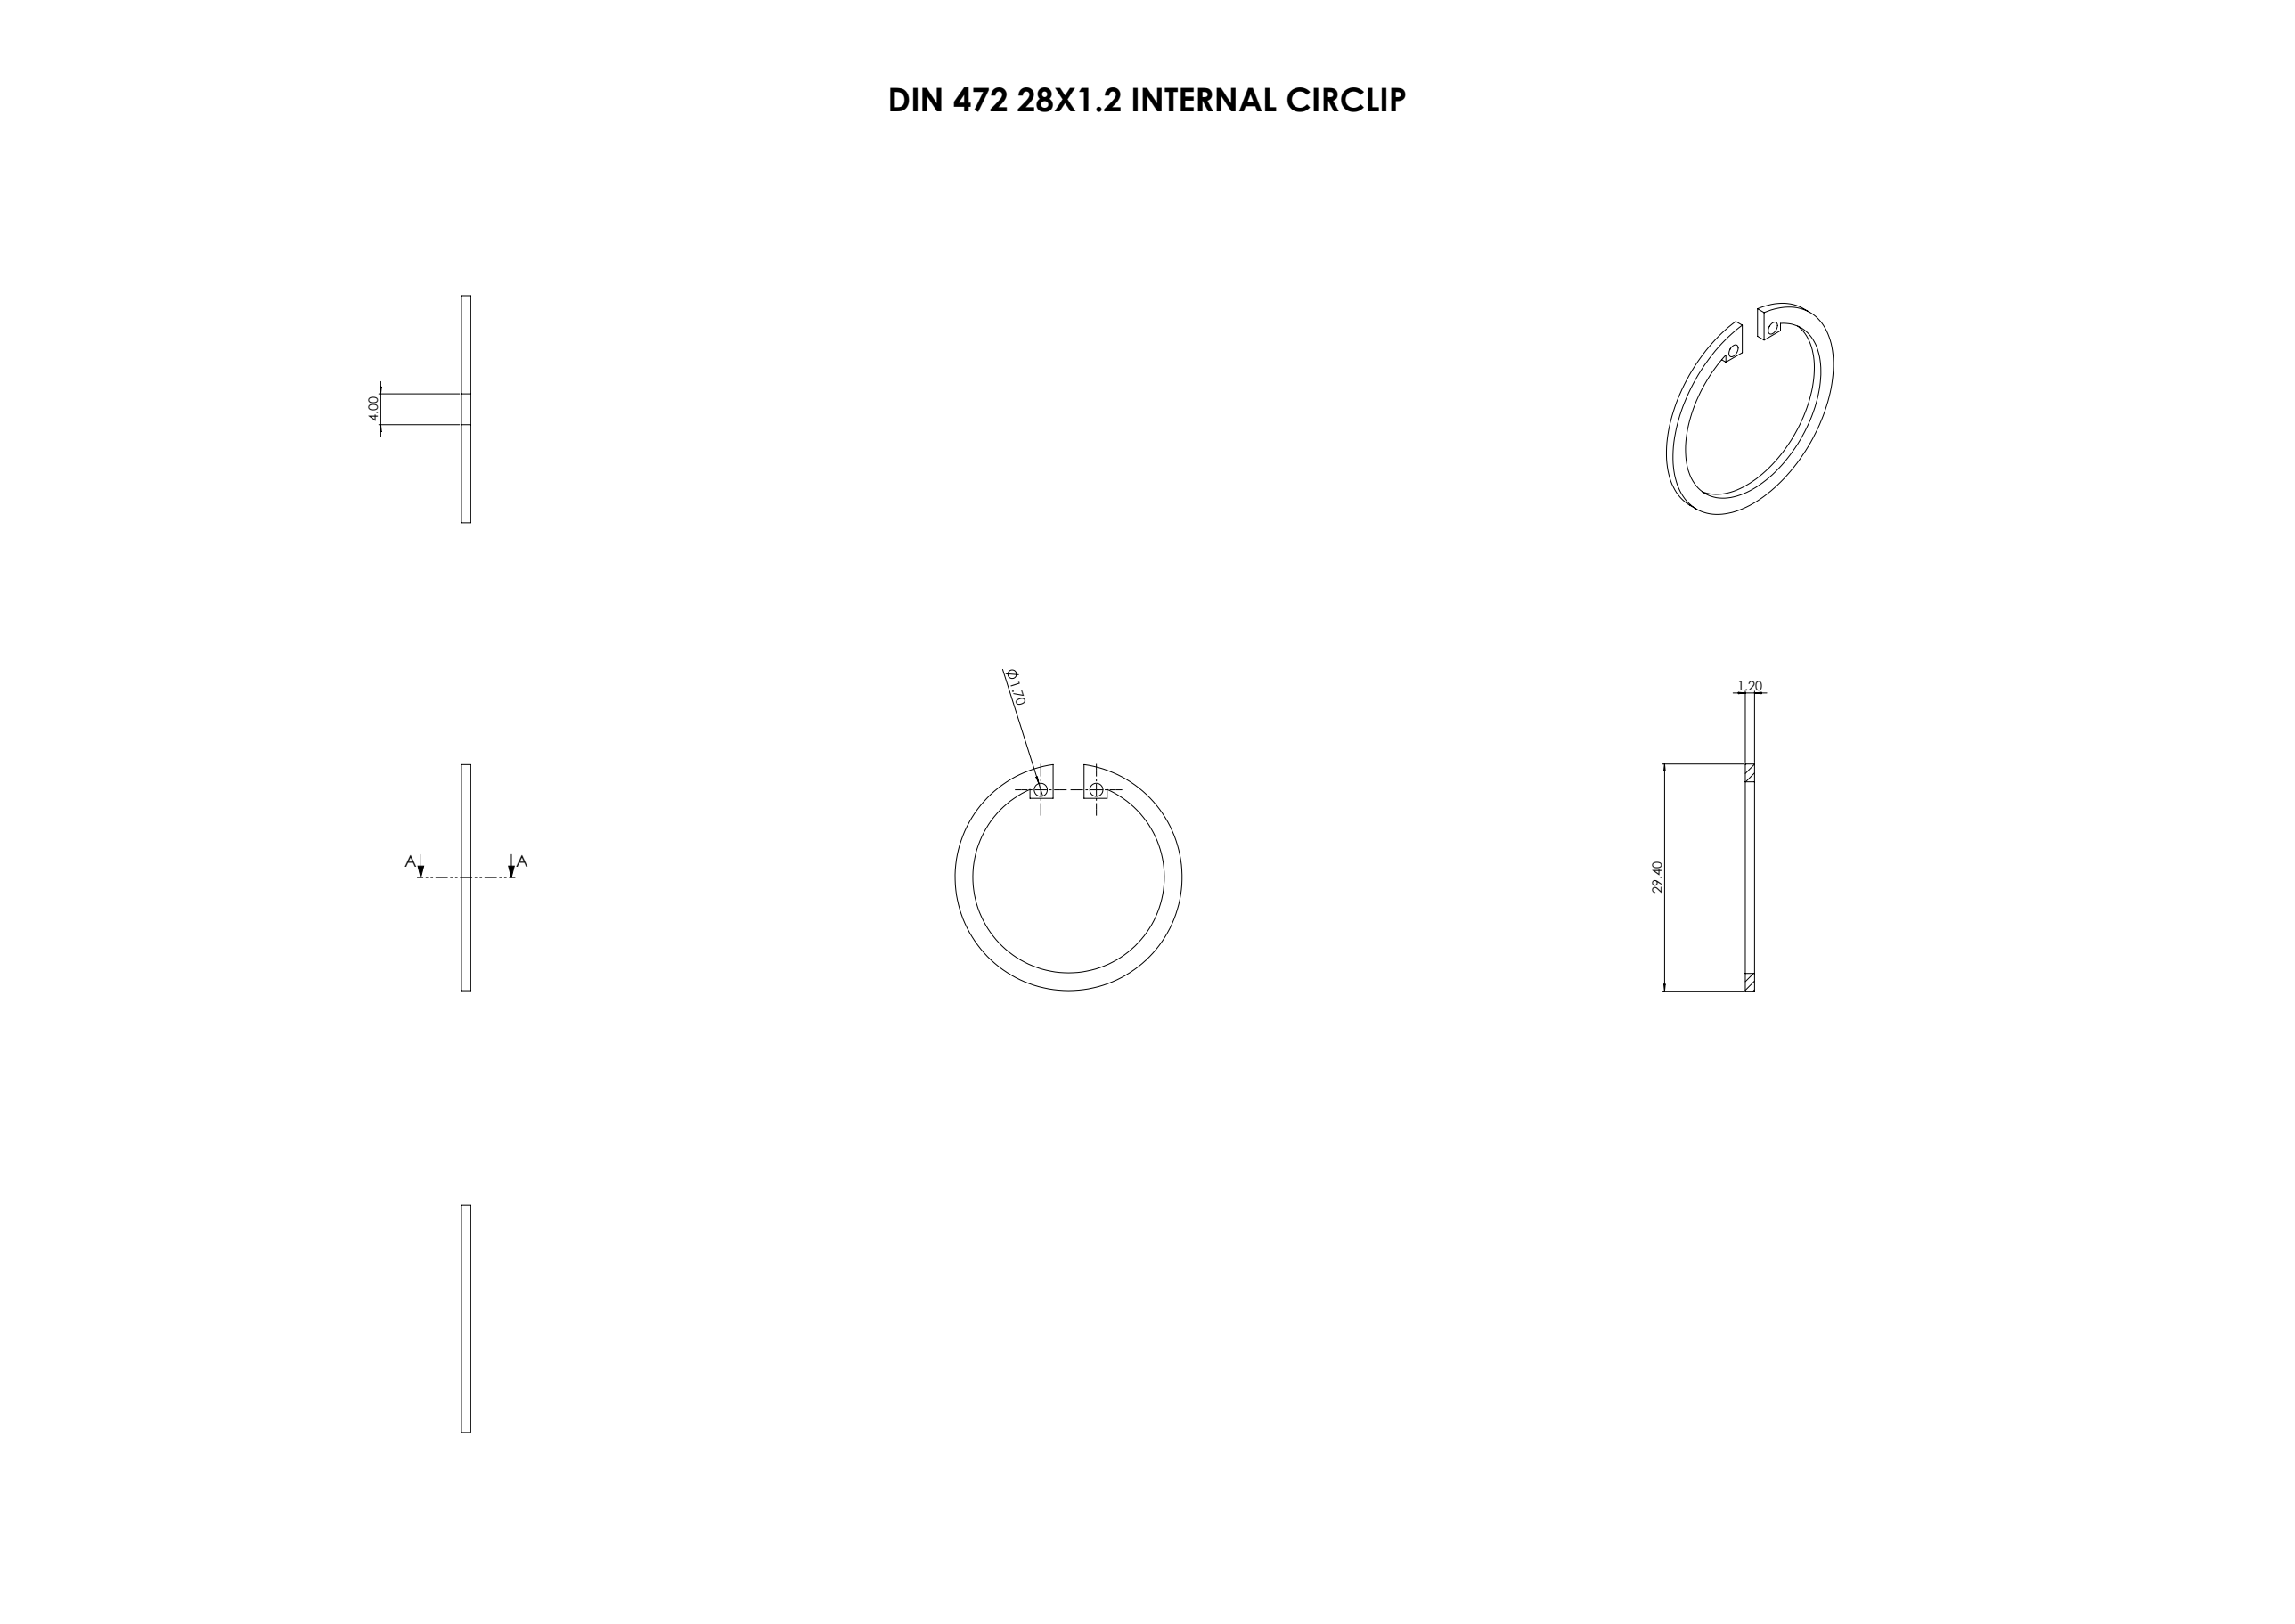
ISO-10303-21;
HEADER;
/* Generated by software containing ST-Developer
 * from STEP Tools, Inc. (www.steptools.com) 
 */

FILE_DESCRIPTION(
/* description */ (''),
/* implementation_level */ '2;1');

FILE_NAME(
/* name */ '10_DIN_472_28x1.2_Internal_Circlip.step',
/* time_stamp */ '2026-10-11T09:12:28-07:00',
/* author */ (''),
/* organization */ (''),
/* preprocessor_version */ 'ST-DEVELOPER v20.2',
/* originating_system */ 'Autodesk Translation Framework v15.15.0.0',
/* authorisation */ '');

FILE_SCHEMA (('AUTOMOTIVE_DESIGN { 1 0 10303 214 3 1 1 }'));
ENDSEC;

DATA;
#10=MECHANICAL_DESIGN_GEOMETRIC_PRESENTATION_REPRESENTATION('',(#656),#23254);
#636=SHAPE_REPRESENTATION_RELATIONSHIP('SRR','None',#23309,#646);
#646=ADVANCED_BREP_SHAPE_REPRESENTATION('',(#666),#23253);
#656=STYLED_ITEM('',(#23462),#666);
#666=MANIFOLD_SOLID_BREP('Body1',#7034);
#848=FACE_BOUND('',#1829,.T.);
#849=FACE_BOUND('',#1830,.T.);
#850=FACE_BOUND('',#1838,.T.);
#851=FACE_BOUND('',#1839,.T.);
#971=PLANE('',#7802);
#972=PLANE('',#7804);
#973=PLANE('',#7805);
#974=PLANE('',#7806);
#975=PLANE('',#7807);
#976=PLANE('',#7808);
#977=PLANE('',#7809);
#978=PLANE('',#7810);
#1362=FACE_OUTER_BOUND('',#1825,.T.);
#1363=FACE_OUTER_BOUND('',#1826,.T.);
#1364=FACE_OUTER_BOUND('',#1827,.T.);
#1365=FACE_OUTER_BOUND('',#1828,.T.);
#1366=FACE_OUTER_BOUND('',#1831,.T.);
#1367=FACE_OUTER_BOUND('',#1832,.T.);
#1368=FACE_OUTER_BOUND('',#1833,.T.);
#1369=FACE_OUTER_BOUND('',#1834,.T.);
#1370=FACE_OUTER_BOUND('',#1835,.T.);
#1371=FACE_OUTER_BOUND('',#1836,.T.);
#1372=FACE_OUTER_BOUND('',#1837,.T.);
#1373=FACE_OUTER_BOUND('',#1840,.T.);
#1825=EDGE_LOOP('',(#6507,#6508,#6509,#6510));
#1826=EDGE_LOOP('',(#6511,#6512,#6513,#6514));
#1827=EDGE_LOOP('',(#6515,#6516,#6517,#6518));
#1828=EDGE_LOOP('',(#6519,#6520,#6521,#6522,#6523,#6524,#6525,#6526));
#1829=EDGE_LOOP('',(#6527));
#1830=EDGE_LOOP('',(#6528));
#1831=EDGE_LOOP('',(#6529,#6530,#6531,#6532));
#1832=EDGE_LOOP('',(#6533,#6534,#6535,#6536));
#1833=EDGE_LOOP('',(#6537,#6538,#6539,#6540));
#1834=EDGE_LOOP('',(#6541,#6542,#6543,#6544));
#1835=EDGE_LOOP('',(#6545,#6546,#6547,#6548));
#1836=EDGE_LOOP('',(#6549,#6550,#6551,#6552));
#1837=EDGE_LOOP('',(#6553,#6554,#6555,#6556,#6557,#6558,#6559,#6560));
#1838=EDGE_LOOP('',(#6561));
#1839=EDGE_LOOP('',(#6562));
#1840=EDGE_LOOP('',(#6563,#6564,#6565,#6566));
#2078=LINE('',#23155,#2337);
#2079=LINE('',#23161,#2338);
#2080=LINE('',#23166,#2339);
#2081=LINE('',#23170,#2340);
#2082=LINE('',#23174,#2341);
#2083=LINE('',#23176,#2342);
#2084=LINE('',#23178,#2343);
#2085=LINE('',#23182,#2344);
#2086=LINE('',#23184,#2345);
#2087=LINE('',#23185,#2346);
#2088=LINE('',#23188,#2347);
#2089=LINE('',#23190,#2348);
#2090=LINE('',#23191,#2349);
#2091=LINE('',#23194,#2350);
#2092=LINE('',#23195,#2351);
#2093=LINE('',#23197,#2352);
#2094=LINE('',#23200,#2353);
#2095=LINE('',#23201,#2354);
#2096=LINE('',#23204,#2355);
#2097=LINE('',#23206,#2356);
#2098=LINE('',#23207,#2357);
#2099=LINE('',#23209,#2358);
#2337=VECTOR('',#9366,0.85);
#2338=VECTOR('',#9373,0.85);
#2339=VECTOR('',#9378,10.);
#2340=VECTOR('',#9381,10.);
#2341=VECTOR('',#9386,10.);
#2342=VECTOR('',#9387,10.);
#2343=VECTOR('',#9388,10.);
#2344=VECTOR('',#9391,10.);
#2345=VECTOR('',#9392,10.);
#2346=VECTOR('',#9393,10.);
#2347=VECTOR('',#9396,10.);
#2348=VECTOR('',#9397,10.);
#2349=VECTOR('',#9398,10.);
#2350=VECTOR('',#9401,10.);
#2351=VECTOR('',#9402,10.);
#2352=VECTOR('',#9405,10.);
#2353=VECTOR('',#9408,10.);
#2354=VECTOR('',#9409,10.);
#2355=VECTOR('',#9412,10.);
#2356=VECTOR('',#9413,10.);
#2357=VECTOR('',#9414,10.);
#2358=VECTOR('',#9417,10.);
#2694=CIRCLE('',#7794,0.85);
#2695=CIRCLE('',#7795,0.85);
#2696=CIRCLE('',#7797,0.85);
#2697=CIRCLE('',#7798,0.85);
#2698=CIRCLE('',#7800,14.7);
#2699=CIRCLE('',#7801,14.7);
#2700=CIRCLE('',#7803,12.4);
#2701=CIRCLE('',#7811,12.4);
#3385=VERTEX_POINT('',#23152);
#3386=VERTEX_POINT('',#23154);
#3387=VERTEX_POINT('',#23158);
#3388=VERTEX_POINT('',#23160);
#3389=VERTEX_POINT('',#23164);
#3390=VERTEX_POINT('',#23165);
#3391=VERTEX_POINT('',#23167);
#3392=VERTEX_POINT('',#23169);
#3393=VERTEX_POINT('',#23173);
#3394=VERTEX_POINT('',#23175);
#3395=VERTEX_POINT('',#23177);
#3396=VERTEX_POINT('',#23179);
#3397=VERTEX_POINT('',#23181);
#3398=VERTEX_POINT('',#23183);
#3399=VERTEX_POINT('',#23187);
#3400=VERTEX_POINT('',#23189);
#3401=VERTEX_POINT('',#23193);
#3402=VERTEX_POINT('',#23199);
#3403=VERTEX_POINT('',#23203);
#3404=VERTEX_POINT('',#23205);
#4429=EDGE_CURVE('',#3385,#3385,#2694,.T.);
#4430=EDGE_CURVE('',#3385,#3386,#2078,.T.);
#4431=EDGE_CURVE('',#3386,#3386,#2695,.T.);
#4432=EDGE_CURVE('',#3387,#3387,#2696,.T.);
#4433=EDGE_CURVE('',#3387,#3388,#2079,.T.);
#4434=EDGE_CURVE('',#3388,#3388,#2697,.T.);
#4435=EDGE_CURVE('',#3389,#3390,#2080,.T.);
#4436=EDGE_CURVE('',#3390,#3391,#2698,.T.);
#4437=EDGE_CURVE('',#3391,#3392,#2081,.T.);
#4438=EDGE_CURVE('',#3389,#3392,#2699,.T.);
#4439=EDGE_CURVE('',#3393,#3390,#2082,.T.);
#4440=EDGE_CURVE('',#3394,#3393,#2083,.T.);
#4441=EDGE_CURVE('',#3395,#3394,#2084,.T.);
#4442=EDGE_CURVE('',#3395,#3396,#2700,.T.);
#4443=EDGE_CURVE('',#3396,#3397,#2085,.T.);
#4444=EDGE_CURVE('',#3397,#3398,#2086,.T.);
#4445=EDGE_CURVE('',#3398,#3391,#2087,.T.);
#4446=EDGE_CURVE('',#3399,#3396,#2088,.T.);
#4447=EDGE_CURVE('',#3400,#3399,#2089,.T.);
#4448=EDGE_CURVE('',#3397,#3400,#2090,.T.);
#4449=EDGE_CURVE('',#3401,#3400,#2091,.T.);
#4450=EDGE_CURVE('',#3398,#3401,#2092,.T.);
#4451=EDGE_CURVE('',#3392,#3401,#2093,.T.);
#4452=EDGE_CURVE('',#3402,#3389,#2094,.T.);
#4453=EDGE_CURVE('',#3393,#3402,#2095,.T.);
#4454=EDGE_CURVE('',#3395,#3403,#2096,.T.);
#4455=EDGE_CURVE('',#3394,#3404,#2097,.T.);
#4456=EDGE_CURVE('',#3403,#3404,#2098,.T.);
#4457=EDGE_CURVE('',#3404,#3402,#2099,.T.);
#4458=EDGE_CURVE('',#3403,#3399,#2701,.T.);
#6507=ORIENTED_EDGE('',*,*,#4429,.F.);
#6508=ORIENTED_EDGE('',*,*,#4430,.T.);
#6509=ORIENTED_EDGE('',*,*,#4431,.F.);
#6510=ORIENTED_EDGE('',*,*,#4430,.F.);
#6511=ORIENTED_EDGE('',*,*,#4432,.F.);
#6512=ORIENTED_EDGE('',*,*,#4433,.T.);
#6513=ORIENTED_EDGE('',*,*,#4434,.F.);
#6514=ORIENTED_EDGE('',*,*,#4433,.F.);
#6515=ORIENTED_EDGE('',*,*,#4435,.T.);
#6516=ORIENTED_EDGE('',*,*,#4436,.T.);
#6517=ORIENTED_EDGE('',*,*,#4437,.T.);
#6518=ORIENTED_EDGE('',*,*,#4438,.F.);
#6519=ORIENTED_EDGE('',*,*,#4439,.F.);
#6520=ORIENTED_EDGE('',*,*,#4440,.F.);
#6521=ORIENTED_EDGE('',*,*,#4441,.F.);
#6522=ORIENTED_EDGE('',*,*,#4442,.T.);
#6523=ORIENTED_EDGE('',*,*,#4443,.T.);
#6524=ORIENTED_EDGE('',*,*,#4444,.T.);
#6525=ORIENTED_EDGE('',*,*,#4445,.T.);
#6526=ORIENTED_EDGE('',*,*,#4436,.F.);
#6527=ORIENTED_EDGE('',*,*,#4432,.T.);
#6528=ORIENTED_EDGE('',*,*,#4429,.T.);
#6529=ORIENTED_EDGE('',*,*,#4446,.F.);
#6530=ORIENTED_EDGE('',*,*,#4447,.F.);
#6531=ORIENTED_EDGE('',*,*,#4448,.F.);
#6532=ORIENTED_EDGE('',*,*,#4443,.F.);
#6533=ORIENTED_EDGE('',*,*,#4444,.F.);
#6534=ORIENTED_EDGE('',*,*,#4448,.T.);
#6535=ORIENTED_EDGE('',*,*,#4449,.F.);
#6536=ORIENTED_EDGE('',*,*,#4450,.F.);
#6537=ORIENTED_EDGE('',*,*,#4445,.F.);
#6538=ORIENTED_EDGE('',*,*,#4450,.T.);
#6539=ORIENTED_EDGE('',*,*,#4451,.F.);
#6540=ORIENTED_EDGE('',*,*,#4437,.F.);
#6541=ORIENTED_EDGE('',*,*,#4452,.F.);
#6542=ORIENTED_EDGE('',*,*,#4453,.F.);
#6543=ORIENTED_EDGE('',*,*,#4439,.T.);
#6544=ORIENTED_EDGE('',*,*,#4435,.F.);
#6545=ORIENTED_EDGE('',*,*,#4454,.F.);
#6546=ORIENTED_EDGE('',*,*,#4441,.T.);
#6547=ORIENTED_EDGE('',*,*,#4455,.T.);
#6548=ORIENTED_EDGE('',*,*,#4456,.F.);
#6549=ORIENTED_EDGE('',*,*,#4440,.T.);
#6550=ORIENTED_EDGE('',*,*,#4453,.T.);
#6551=ORIENTED_EDGE('',*,*,#4457,.F.);
#6552=ORIENTED_EDGE('',*,*,#4455,.F.);
#6553=ORIENTED_EDGE('',*,*,#4452,.T.);
#6554=ORIENTED_EDGE('',*,*,#4438,.T.);
#6555=ORIENTED_EDGE('',*,*,#4451,.T.);
#6556=ORIENTED_EDGE('',*,*,#4449,.T.);
#6557=ORIENTED_EDGE('',*,*,#4447,.T.);
#6558=ORIENTED_EDGE('',*,*,#4458,.F.);
#6559=ORIENTED_EDGE('',*,*,#4456,.T.);
#6560=ORIENTED_EDGE('',*,*,#4457,.T.);
#6561=ORIENTED_EDGE('',*,*,#4431,.T.);
#6562=ORIENTED_EDGE('',*,*,#4434,.T.);
#6563=ORIENTED_EDGE('',*,*,#4446,.T.);
#6564=ORIENTED_EDGE('',*,*,#4442,.F.);
#6565=ORIENTED_EDGE('',*,*,#4454,.T.);
#6566=ORIENTED_EDGE('',*,*,#4458,.T.);
#6626=CYLINDRICAL_SURFACE('',#7793,0.85);
#6627=CYLINDRICAL_SURFACE('',#7796,0.85);
#6628=CYLINDRICAL_SURFACE('',#7799,14.7);
#6629=CYLINDRICAL_SURFACE('',#7812,12.4);
#7013=ADVANCED_FACE('',(#1362),#6626,.F.);
#7014=ADVANCED_FACE('',(#1363),#6627,.F.);
#7015=ADVANCED_FACE('',(#1364),#6628,.T.);
#7016=ADVANCED_FACE('',(#1365,#848,#849),#971,.T.);
#7017=ADVANCED_FACE('',(#1366),#972,.T.);
#7018=ADVANCED_FACE('',(#1367),#973,.T.);
#7019=ADVANCED_FACE('',(#1368),#974,.T.);
#7020=ADVANCED_FACE('',(#1369),#975,.T.);
#7021=ADVANCED_FACE('',(#1370),#976,.T.);
#7022=ADVANCED_FACE('',(#1371),#977,.T.);
#7023=ADVANCED_FACE('',(#1372,#850,#851),#978,.T.);
#7024=ADVANCED_FACE('',(#1373),#6629,.F.);
#7034=CLOSED_SHELL('',(#7013,#7014,#7015,#7016,#7017,#7018,#7019,#7020,
#7021,#7022,#7023,#7024));
#7792=AXIS2_PLACEMENT_3D('',#23150,#9360,#9361);
#7793=AXIS2_PLACEMENT_3D('',#23151,#9362,#9363);
#7794=AXIS2_PLACEMENT_3D('',#23153,#9364,#9365);
#7795=AXIS2_PLACEMENT_3D('',#23156,#9367,#9368);
#7796=AXIS2_PLACEMENT_3D('',#23157,#9369,#9370);
#7797=AXIS2_PLACEMENT_3D('',#23159,#9371,#9372);
#7798=AXIS2_PLACEMENT_3D('',#23162,#9374,#9375);
#7799=AXIS2_PLACEMENT_3D('',#23163,#9376,#9377);
#7800=AXIS2_PLACEMENT_3D('',#23168,#9379,#9380);
#7801=AXIS2_PLACEMENT_3D('',#23171,#9382,#9383);
#7802=AXIS2_PLACEMENT_3D('',#23172,#9384,#9385);
#7803=AXIS2_PLACEMENT_3D('',#23180,#9389,#9390);
#7804=AXIS2_PLACEMENT_3D('',#23186,#9394,#9395);
#7805=AXIS2_PLACEMENT_3D('',#23192,#9399,#9400);
#7806=AXIS2_PLACEMENT_3D('',#23196,#9403,#9404);
#7807=AXIS2_PLACEMENT_3D('',#23198,#9406,#9407);
#7808=AXIS2_PLACEMENT_3D('',#23202,#9410,#9411);
#7809=AXIS2_PLACEMENT_3D('',#23208,#9415,#9416);
#7810=AXIS2_PLACEMENT_3D('',#23210,#9418,#9419);
#7811=AXIS2_PLACEMENT_3D('',#23211,#9420,#9421);
#7812=AXIS2_PLACEMENT_3D('',#23212,#9422,#9423);
#9360=DIRECTION('axis',(0.,0.,1.));
#9361=DIRECTION('refdir',(1.,0.,0.));
#9362=DIRECTION('center_axis',(1.,0.,0.));
#9363=DIRECTION('ref_axis',(0.,0.,-1.));
#9364=DIRECTION('center_axis',(1.,0.,0.));
#9365=DIRECTION('ref_axis',(0.,0.,-1.));
#9366=DIRECTION('',(1.,0.,0.));
#9367=DIRECTION('center_axis',(-1.,0.,0.));
#9368=DIRECTION('ref_axis',(0.,0.,-1.));
#9369=DIRECTION('center_axis',(1.,0.,0.));
#9370=DIRECTION('ref_axis',(0.,0.,-1.));
#9371=DIRECTION('center_axis',(1.,0.,0.));
#9372=DIRECTION('ref_axis',(0.,0.,-1.));
#9373=DIRECTION('',(1.,0.,0.));
#9374=DIRECTION('center_axis',(-1.,0.,0.));
#9375=DIRECTION('ref_axis',(0.,0.,-1.));
#9376=DIRECTION('center_axis',(1.,0.,0.));
#9377=DIRECTION('ref_axis',(0.,-1.,1.22464679914735E-16));
#9378=DIRECTION('',(-1.,0.,0.));
#9379=DIRECTION('center_axis',(1.,0.,0.));
#9380=DIRECTION('ref_axis',(0.,0.,-1.));
#9381=DIRECTION('',(1.,0.,0.));
#9382=DIRECTION('center_axis',(1.,0.,0.));
#9383=DIRECTION('ref_axis',(0.,0.,-1.));
#9384=DIRECTION('center_axis',(-1.,0.,0.));
#9385=DIRECTION('ref_axis',(0.,0.,1.));
#9386=DIRECTION('',(0.,1.,0.));
#9387=DIRECTION('',(0.,0.,-1.));
#9388=DIRECTION('',(0.,-1.,0.));
#9389=DIRECTION('center_axis',(1.,0.,0.));
#9390=DIRECTION('ref_axis',(0.,0.,-1.));
#9391=DIRECTION('',(0.,-1.,0.));
#9392=DIRECTION('',(0.,0.,1.));
#9393=DIRECTION('',(0.,1.,0.));
#9394=DIRECTION('center_axis',(0.,0.,-1.));
#9395=DIRECTION('ref_axis',(0.,1.,0.));
#9396=DIRECTION('',(-1.,0.,0.));
#9397=DIRECTION('',(0.,1.,0.));
#9398=DIRECTION('',(1.,0.,0.));
#9399=DIRECTION('center_axis',(0.,-1.,0.));
#9400=DIRECTION('ref_axis',(0.,0.,-1.));
#9401=DIRECTION('',(0.,0.,-1.));
#9402=DIRECTION('',(1.,0.,0.));
#9403=DIRECTION('center_axis',(0.,0.,1.));
#9404=DIRECTION('ref_axis',(0.,-1.,0.));
#9405=DIRECTION('',(0.,-1.,0.));
#9406=DIRECTION('center_axis',(0.,0.,-1.));
#9407=DIRECTION('ref_axis',(0.,1.,0.));
#9408=DIRECTION('',(0.,1.,0.));
#9409=DIRECTION('',(1.,0.,0.));
#9410=DIRECTION('center_axis',(0.,0.,1.));
#9411=DIRECTION('ref_axis',(0.,-1.,0.));
#9412=DIRECTION('',(1.,0.,0.));
#9413=DIRECTION('',(1.,0.,0.));
#9414=DIRECTION('',(0.,-1.,0.));
#9415=DIRECTION('center_axis',(0.,-1.,0.));
#9416=DIRECTION('ref_axis',(0.,0.,-1.));
#9417=DIRECTION('',(0.,0.,-1.));
#9418=DIRECTION('center_axis',(1.,0.,0.));
#9419=DIRECTION('ref_axis',(0.,0.,-1.));
#9420=DIRECTION('center_axis',(1.,0.,0.));
#9421=DIRECTION('ref_axis',(0.,0.,-1.));
#9422=DIRECTION('center_axis',(1.,0.,0.));
#9423=DIRECTION('ref_axis',(0.,-1.,-1.22464679914735E-16));
#23150=CARTESIAN_POINT('',(0.,0.,0.));
#23151=CARTESIAN_POINT('Origin',(0.,11.3,3.6));
#23152=CARTESIAN_POINT('',(0.,11.3,4.45));
#23153=CARTESIAN_POINT('Origin',(0.,11.3,3.6));
#23154=CARTESIAN_POINT('',(1.2,11.3,4.45));
#23155=CARTESIAN_POINT('',(0.,11.3,4.45));
#23156=CARTESIAN_POINT('Origin',(1.2,11.3,3.6));
#23157=CARTESIAN_POINT('Origin',(0.,11.3,-3.6));
#23158=CARTESIAN_POINT('',(0.,11.3,-2.75));
#23159=CARTESIAN_POINT('Origin',(0.,11.3,-3.6));
#23160=CARTESIAN_POINT('',(1.2,11.3,-2.75));
#23161=CARTESIAN_POINT('',(0.,11.3,-2.75));
#23162=CARTESIAN_POINT('Origin',(1.2,11.3,-3.6));
#23163=CARTESIAN_POINT('Origin',(0.6,0.,0.));
#23164=CARTESIAN_POINT('',(1.2,14.5633100633063,2.));
#23165=CARTESIAN_POINT('',(0.,14.5633100633063,2.));
#23166=CARTESIAN_POINT('',(0.6,14.5633100633063,2.));
#23167=CARTESIAN_POINT('',(0.,14.5633100633063,-2.));
#23168=CARTESIAN_POINT('Origin',(0.,0.,0.));
#23169=CARTESIAN_POINT('',(1.2,14.5633100633063,-2.));
#23170=CARTESIAN_POINT('',(0.6,14.5633100633063,-2.));
#23171=CARTESIAN_POINT('Origin',(1.2,0.,0.));
#23172=CARTESIAN_POINT('Origin',(0.,14.7,0.));
#23173=CARTESIAN_POINT('',(0.,10.2,2.));
#23174=CARTESIAN_POINT('',(0.,10.2,2.));
#23175=CARTESIAN_POINT('',(0.,10.2,5.));
#23176=CARTESIAN_POINT('',(0.,10.2,5.));
#23177=CARTESIAN_POINT('',(0.,11.3472463620034,5.));
#23178=CARTESIAN_POINT('',(0.,12.6,5.));
#23179=CARTESIAN_POINT('',(0.,11.3472463620034,-5.));
#23180=CARTESIAN_POINT('Origin',(0.,0.,0.));
#23181=CARTESIAN_POINT('',(0.,10.2,-5.));
#23182=CARTESIAN_POINT('',(0.,12.6,-5.));
#23183=CARTESIAN_POINT('',(0.,10.2,-2.));
#23184=CARTESIAN_POINT('',(0.,10.2,-5.));
#23185=CARTESIAN_POINT('',(0.,12.1,-2.));
#23186=CARTESIAN_POINT('Origin',(0.,10.2,-5.));
#23187=CARTESIAN_POINT('',(1.2,11.3472463620034,-5.));
#23188=CARTESIAN_POINT('',(0.6,11.3472463620034,-5.));
#23189=CARTESIAN_POINT('',(1.2,10.2,-5.));
#23190=CARTESIAN_POINT('',(1.2,12.6,-5.));
#23191=CARTESIAN_POINT('',(0.,10.2,-5.));
#23192=CARTESIAN_POINT('Origin',(0.,10.2,-2.));
#23193=CARTESIAN_POINT('',(1.2,10.2,-2.));
#23194=CARTESIAN_POINT('',(1.2,10.2,-5.));
#23195=CARTESIAN_POINT('',(0.,10.2,-2.));
#23196=CARTESIAN_POINT('Origin',(0.,12.6,-2.));
#23197=CARTESIAN_POINT('',(1.2,10.95,-2.));
#23198=CARTESIAN_POINT('Origin',(0.,10.2,2.));
#23199=CARTESIAN_POINT('',(1.2,10.2,2.));
#23200=CARTESIAN_POINT('',(1.2,13.95,2.));
#23201=CARTESIAN_POINT('',(0.,10.2,2.));
#23202=CARTESIAN_POINT('Origin',(0.,12.6,5.));
#23203=CARTESIAN_POINT('',(1.2,11.3472463620034,5.));
#23204=CARTESIAN_POINT('',(0.6,11.3472463620034,5.));
#23205=CARTESIAN_POINT('',(1.2,10.2,5.));
#23206=CARTESIAN_POINT('',(0.,10.2,5.));
#23207=CARTESIAN_POINT('',(1.2,12.6,5.));
#23208=CARTESIAN_POINT('Origin',(0.,10.2,5.));
#23209=CARTESIAN_POINT('',(1.2,10.2,5.));
#23210=CARTESIAN_POINT('Origin',(1.2,12.4,0.));
#23211=CARTESIAN_POINT('Origin',(1.2,0.,0.));
#23212=CARTESIAN_POINT('Origin',(0.6,0.,0.));
#23241=UNCERTAINTY_MEASURE_WITH_UNIT(LENGTH_MEASURE(0.01),#23255,
'DISTANCE_ACCURACY_VALUE',
'Maximum model space distance between geometric entities at asserted c
onnectivities');
#23242=UNCERTAINTY_MEASURE_WITH_UNIT(LENGTH_MEASURE(0.01),#23255,
'DISTANCE_ACCURACY_VALUE',
'Maximum model space distance between geometric entities at asserted c
onnectivities');
#23253=(
GEOMETRIC_REPRESENTATION_CONTEXT(3)
GLOBAL_UNCERTAINTY_ASSIGNED_CONTEXT((#23241))
GLOBAL_UNIT_ASSIGNED_CONTEXT((#23255,#23257,#23258))
REPRESENTATION_CONTEXT('','3D')
);
#23254=(
GEOMETRIC_REPRESENTATION_CONTEXT(3)
GLOBAL_UNCERTAINTY_ASSIGNED_CONTEXT((#23242))
GLOBAL_UNIT_ASSIGNED_CONTEXT((#23255,#23257,#23258))
REPRESENTATION_CONTEXT('','3D')
);
#23255=(
LENGTH_UNIT()
NAMED_UNIT(*)
SI_UNIT(.MILLI.,.METRE.)
);
#23257=(
NAMED_UNIT(*)
PLANE_ANGLE_UNIT()
SI_UNIT($,.RADIAN.)
);
#23258=(
NAMED_UNIT(*)
SI_UNIT($,.STERADIAN.)
SOLID_ANGLE_UNIT()
);
#23269=SHAPE_DEFINITION_REPRESENTATION(#23280,#23309);
#23280=PRODUCT_DEFINITION_SHAPE('',$,#23321);
#23309=SHAPE_REPRESENTATION('',(#7792),#23253);
#23310=PRODUCT_DEFINITION_CONTEXT('part definition',#23345,'design');
#23321=PRODUCT_DEFINITION('2026-10-11-09-11-56-293',
'10_DIN_472_28x1.2_Internal_Circlip',#23332,#23310);
#23332=PRODUCT_DEFINITION_FORMATION('',$,#23357);
#23345=APPLICATION_CONTEXT(
'Core Data for Automotive Mechanical Design Process');
#23346=PRODUCT_CONTEXT('part definition',#23345,'mechanical');
#23357=PRODUCT('2026-10-11-09-11-56-293',
'10_DIN_472_28x1.2_Internal_Circlip',$,(#23346));
#23456=COLOUR_RGB('Grey',0.48,0.52,0.57);
#23457=FILL_AREA_STYLE_COLOUR('',#23456);
#23458=FILL_AREA_STYLE('',(#23457));
#23459=SURFACE_STYLE_FILL_AREA(#23458);
#23460=SURFACE_SIDE_STYLE('',(#23459));
#23461=SURFACE_STYLE_USAGE(.BOTH.,#23460);
#23462=PRESENTATION_STYLE_ASSIGNMENT((#23461));
ENDSEC;
END-ISO-10303-21;
